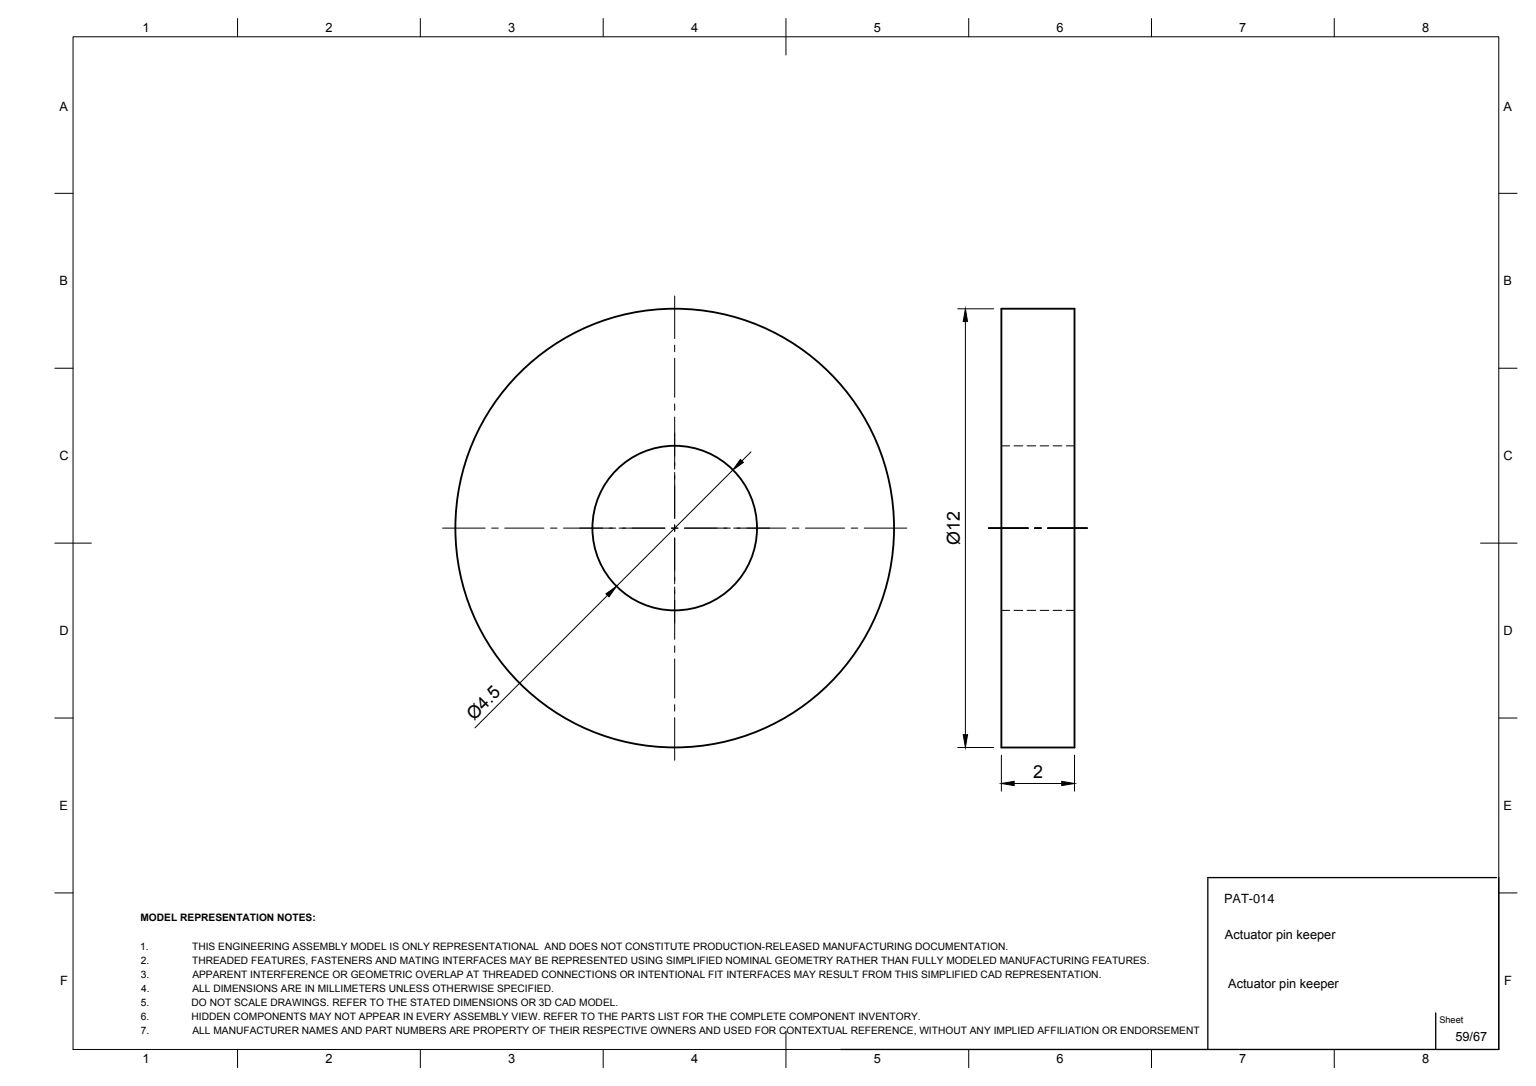
ISO-10303-21;
HEADER;
/* Generated by software containing ST-Developer
 * from STEP Tools, Inc. (www.steptools.com) 
 */

FILE_DESCRIPTION(
/* description */ ('Bin tilter linkage'),
/* implementation_level */ '2;1');

FILE_NAME(
/* name */ 'Actuator pin keeper.step',
/* time_stamp */ '2026-10-28T03:26:24-07:00',
/* author */ (''),
/* organization */ (''),
/* preprocessor_version */ 'ST-DEVELOPER v20.2',
/* originating_system */ 'Autodesk Translation Framework v15.17.0.0',
/* authorisation */ '');

FILE_SCHEMA (('AUTOMOTIVE_DESIGN { 1 0 10303 214 3 1 1 }'));
ENDSEC;

DATA;
#10=MECHANICAL_DESIGN_GEOMETRIC_PRESENTATION_REPRESENTATION('',(#965),#23728);
#745=SHAPE_REPRESENTATION_RELATIONSHIP('SRR','None',#24214,#851);
#851=ADVANCED_BREP_SHAPE_REPRESENTATION('',(#1077),#23714);
#965=STYLED_ITEM('',(#24765),#1077);
#1077=MANIFOLD_SOLID_BREP('Body1',#12497);
#1466=FACE_BOUND('',#3751,.T.);
#1467=FACE_BOUND('',#3753,.T.);
#1844=PLANE('',#15306);
#1845=PLANE('',#15307);
#2592=FACE_OUTER_BOUND('',#3748,.T.);
#2593=FACE_OUTER_BOUND('',#3749,.T.);
#2594=FACE_OUTER_BOUND('',#3750,.T.);
#2595=FACE_OUTER_BOUND('',#3752,.T.);
#3748=EDGE_LOOP('',(#11003,#11004,#11005,#11006));
#3749=EDGE_LOOP('',(#11007,#11008,#11009,#11010));
#3750=EDGE_LOOP('',(#11011));
#3751=EDGE_LOOP('',(#11012));
#3752=EDGE_LOOP('',(#11013));
#3753=EDGE_LOOP('',(#11014));
#4453=LINE('',#23167,#5128);
#4454=LINE('',#23173,#5129);
#5128=VECTOR('',#19330,0.225);
#5129=VECTOR('',#19337,0.6);
#5896=CIRCLE('',#15301,0.225);
#5897=CIRCLE('',#15302,0.225);
#5898=CIRCLE('',#15304,0.6);
#5899=CIRCLE('',#15305,0.6);
#6839=VERTEX_POINT('',#23164);
#6840=VERTEX_POINT('',#23166);
#6841=VERTEX_POINT('',#23170);
#6842=VERTEX_POINT('',#23172);
#8241=EDGE_CURVE('',#6839,#6839,#5896,.T.);
#8242=EDGE_CURVE('',#6839,#6840,#4453,.T.);
#8243=EDGE_CURVE('',#6840,#6840,#5897,.T.);
#8244=EDGE_CURVE('',#6841,#6841,#5898,.T.);
#8245=EDGE_CURVE('',#6841,#6842,#4454,.T.);
#8246=EDGE_CURVE('',#6842,#6842,#5899,.T.);
#11003=ORIENTED_EDGE('',*,*,#8241,.F.);
#11004=ORIENTED_EDGE('',*,*,#8242,.T.);
#11005=ORIENTED_EDGE('',*,*,#8243,.T.);
#11006=ORIENTED_EDGE('',*,*,#8242,.F.);
#11007=ORIENTED_EDGE('',*,*,#8244,.F.);
#11008=ORIENTED_EDGE('',*,*,#8245,.T.);
#11009=ORIENTED_EDGE('',*,*,#8246,.T.);
#11010=ORIENTED_EDGE('',*,*,#8245,.F.);
#11011=ORIENTED_EDGE('',*,*,#8244,.T.);
#11012=ORIENTED_EDGE('',*,*,#8241,.T.);
#11013=ORIENTED_EDGE('',*,*,#8246,.F.);
#11014=ORIENTED_EDGE('',*,*,#8243,.F.);
#11589=CYLINDRICAL_SURFACE('',#15300,0.225);
#11590=CYLINDRICAL_SURFACE('',#15303,0.6);
#12317=ADVANCED_FACE('',(#2592),#11589,.F.);
#12318=ADVANCED_FACE('',(#2593),#11590,.T.);
#12319=ADVANCED_FACE('',(#2594,#1466),#1844,.T.);
#12320=ADVANCED_FACE('',(#2595,#1467),#1845,.F.);
#12497=CLOSED_SHELL('',(#12317,#12318,#12319,#12320));
#15299=AXIS2_PLACEMENT_3D('',#23162,#19324,#19325);
#15300=AXIS2_PLACEMENT_3D('',#23163,#19326,#19327);
#15301=AXIS2_PLACEMENT_3D('',#23165,#19328,#19329);
#15302=AXIS2_PLACEMENT_3D('',#23168,#19331,#19332);
#15303=AXIS2_PLACEMENT_3D('',#23169,#19333,#19334);
#15304=AXIS2_PLACEMENT_3D('',#23171,#19335,#19336);
#15305=AXIS2_PLACEMENT_3D('',#23174,#19338,#19339);
#15306=AXIS2_PLACEMENT_3D('',#23175,#19340,#19341);
#15307=AXIS2_PLACEMENT_3D('',#23176,#19342,#19343);
#19324=DIRECTION('axis',(0.,0.,1.));
#19325=DIRECTION('refdir',(1.,0.,0.));
#19326=DIRECTION('center_axis',(0.,1.,0.));
#19327=DIRECTION('ref_axis',(1.,0.,0.));
#19328=DIRECTION('center_axis',(0.,-1.,0.));
#19329=DIRECTION('ref_axis',(1.,0.,0.));
#19330=DIRECTION('',(0.,-1.,0.));
#19331=DIRECTION('center_axis',(0.,-1.,0.));
#19332=DIRECTION('ref_axis',(1.,0.,0.));
#19333=DIRECTION('center_axis',(0.,1.,0.));
#19334=DIRECTION('ref_axis',(1.,0.,0.));
#19335=DIRECTION('center_axis',(0.,1.,0.));
#19336=DIRECTION('ref_axis',(1.,0.,0.));
#19337=DIRECTION('',(0.,-1.,0.));
#19338=DIRECTION('center_axis',(0.,1.,0.));
#19339=DIRECTION('ref_axis',(1.,0.,0.));
#19340=DIRECTION('center_axis',(0.,1.,0.));
#19341=DIRECTION('ref_axis',(1.,0.,0.));
#19342=DIRECTION('center_axis',(0.,1.,0.));
#19343=DIRECTION('ref_axis',(1.,0.,0.));
#23162=CARTESIAN_POINT('',(0.,0.,0.));
#23163=CARTESIAN_POINT('Origin',(-4.,-3.,11.));
#23164=CARTESIAN_POINT('',(-4.225,-2.8,11.));
#23165=CARTESIAN_POINT('Origin',(-4.,-2.8,11.));
#23166=CARTESIAN_POINT('',(-4.225,-3.,11.));
#23167=CARTESIAN_POINT('',(-4.225,-3.,11.));
#23168=CARTESIAN_POINT('Origin',(-4.,-3.,11.));
#23169=CARTESIAN_POINT('Origin',(-4.,-3.,11.));
#23170=CARTESIAN_POINT('',(-4.6,-2.8,11.));
#23171=CARTESIAN_POINT('Origin',(-4.,-2.8,11.));
#23172=CARTESIAN_POINT('',(-4.6,-3.,11.));
#23173=CARTESIAN_POINT('',(-4.6,-3.,11.));
#23174=CARTESIAN_POINT('Origin',(-4.,-3.,11.));
#23175=CARTESIAN_POINT('Origin',(-4.,-2.8,11.));
#23176=CARTESIAN_POINT('Origin',(-4.,-3.,11.));
#23597=UNCERTAINTY_MEASURE_WITH_UNIT(LENGTH_MEASURE(0.001),#23729,
'DISTANCE_ACCURACY_VALUE',
'Maximum model space distance between geometric entities at asserted c
onnectivities');
#23611=UNCERTAINTY_MEASURE_WITH_UNIT(LENGTH_MEASURE(0.001),#23729,
'DISTANCE_ACCURACY_VALUE',
'Maximum model space distance between geometric entities at asserted c
onnectivities');
#23714=(
GEOMETRIC_REPRESENTATION_CONTEXT(3)
GLOBAL_UNCERTAINTY_ASSIGNED_CONTEXT((#23597))
GLOBAL_UNIT_ASSIGNED_CONTEXT((#23729,#23731,#23732))
REPRESENTATION_CONTEXT('','3D')
);
#23728=(
GEOMETRIC_REPRESENTATION_CONTEXT(3)
GLOBAL_UNCERTAINTY_ASSIGNED_CONTEXT((#23611))
GLOBAL_UNIT_ASSIGNED_CONTEXT((#23729,#23731,#23732))
REPRESENTATION_CONTEXT('','3D')
);
#23729=(
LENGTH_UNIT()
NAMED_UNIT(*)
SI_UNIT(.CENTI.,.METRE.)
);
#23731=(
NAMED_UNIT(*)
PLANE_ANGLE_UNIT()
SI_UNIT($,.RADIAN.)
);
#23732=(
NAMED_UNIT(*)
SI_UNIT($,.STERADIAN.)
SOLID_ANGLE_UNIT()
);
#23835=SHAPE_DEFINITION_REPRESENTATION(#24073,#24214);
#24073=PRODUCT_DEFINITION_SHAPE('',$,#24331);
#24214=SHAPE_REPRESENTATION('',(#15299),#23714);
#24228=PRODUCT_DEFINITION_CONTEXT('part definition',#24578,'design');
#24331=PRODUCT_DEFINITION('Actuator pin keeper','Actuator pin keeper',#24447,
#24228);
#24447=PRODUCT_DEFINITION_FORMATION('',$,#24682);
#24578=APPLICATION_CONTEXT(
'Core Data for Automotive Mechanical Design Process');
#24579=PRODUCT_CONTEXT('part definition',#24578,'mechanical');
#24682=PRODUCT('Actuator pin keeper','Actuator pin keeper',
'Actuator pin keeper',(#24579));
#24759=COLOUR_RGB('Grey',0.48,0.52,0.57);
#24760=FILL_AREA_STYLE_COLOUR('',#24759);
#24761=FILL_AREA_STYLE('',(#24760));
#24762=SURFACE_STYLE_FILL_AREA(#24761);
#24763=SURFACE_SIDE_STYLE('',(#24762));
#24764=SURFACE_STYLE_USAGE(.BOTH.,#24763);
#24765=PRESENTATION_STYLE_ASSIGNMENT((#24764));
ENDSEC;
END-ISO-10303-21;
